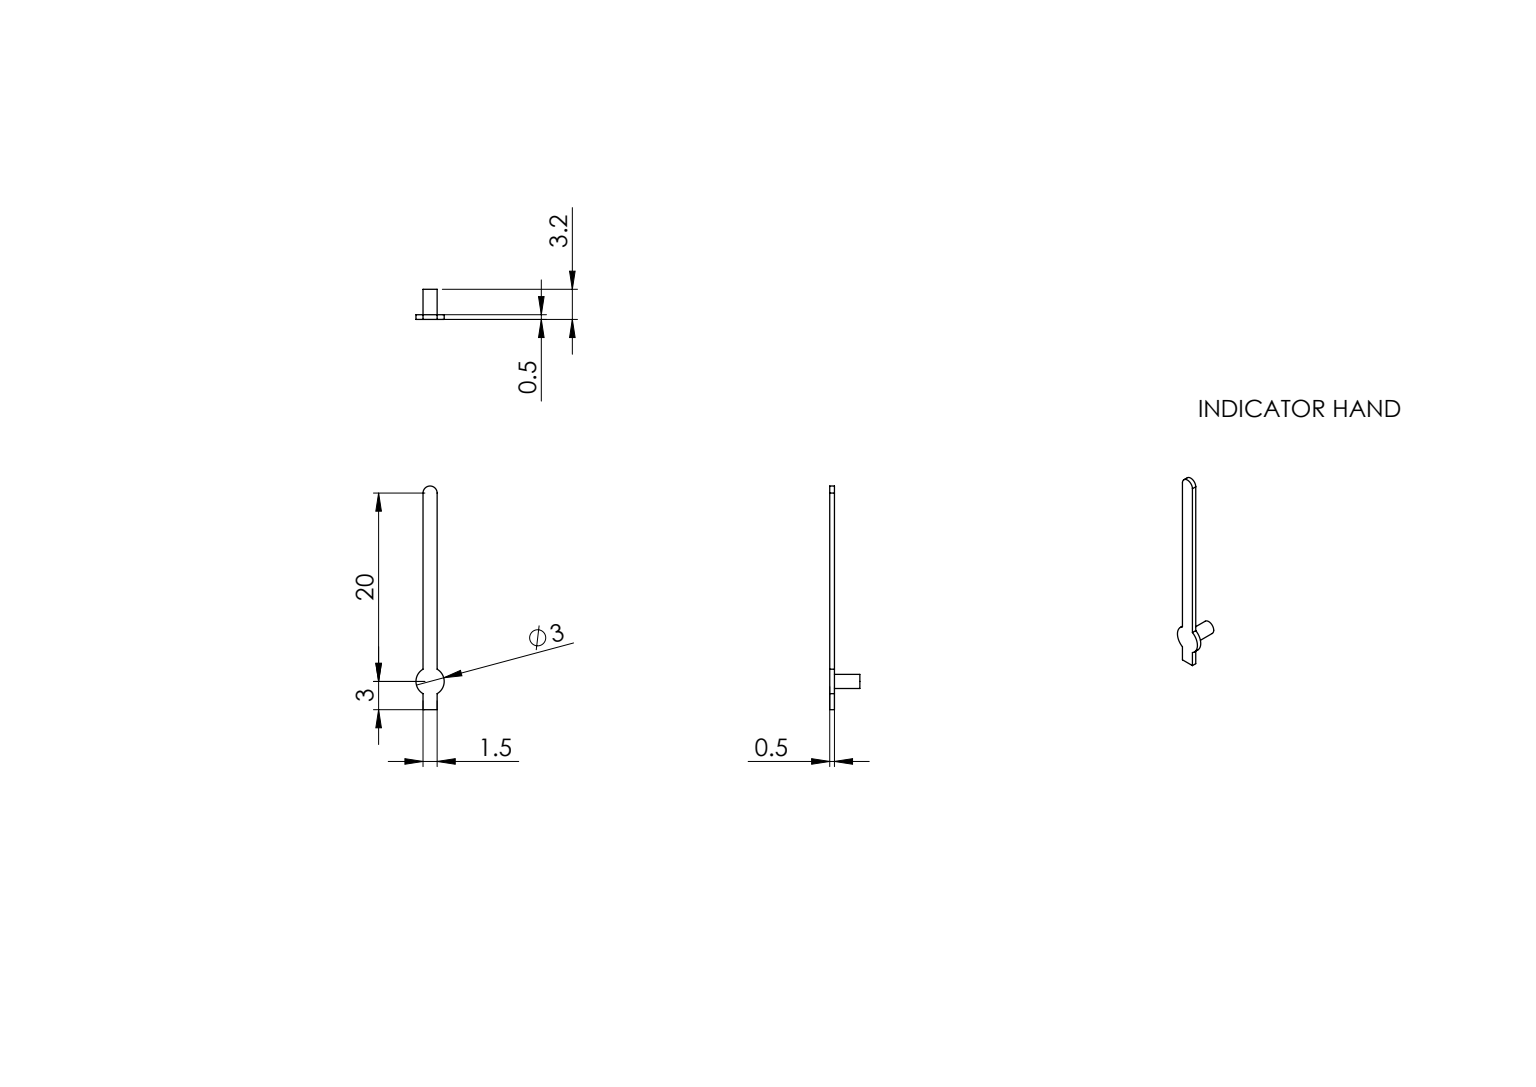
ISO-10303-21;
HEADER;
FILE_DESCRIPTION (('STEP AP214'),
    '1' );
FILE_NAME ('indicator hand.step',
    '2026-10-26T12:50:16',
    ( '' ),
    ( '' ),
    'SwSTEP 2.0',
    'SolidWorks 2026',
    '' );
FILE_SCHEMA (( 'AUTOMOTIVE_DESIGN' ));
ENDSEC;

DATA;
#4=SHAPE_REPRESENTATION_RELATIONSHIP ( 'NONE' , 'NONE' ,  #4483, #7868 ) ;
#16=EDGE_CURVE ( 'NONE', #18357, #14663, #23368, .T. ) ;
#30=CYLINDRICAL_SURFACE ( 'NONE', #8395, 1.500000000000000222 ) ;
#77=( LENGTH_UNIT ( ) NAMED_UNIT ( * ) SI_UNIT ( .MILLI., .METRE. ) );
#128=LINE ( 'NONE', #11881, #5846 ) ;
#265=DIRECTION ( 'NONE',  ( -0.000000000000000000, 0.000000000000000000, 1.000000000000000000 ) ) ;
#311=VERTEX_POINT ( 'NONE', #18646 ) ;
#314=EDGE_CURVE ( 'NONE', #21568, #311, #8696, .T. ) ;
#316=ORIENTED_EDGE ( 'NONE', *, *, #23479, .F. ) ;
#369=ORIENTED_EDGE ( 'NONE', *, *, #4197, .F. ) ;
#391=DIRECTION ( 'NONE',  ( 0.000000000000000000, 0.000000000000000000, -1.000000000000000000 ) ) ;
#413=CIRCLE ( 'NONE', #7088, 1.500000000000000222 ) ;
#423=LINE ( 'NONE', #3954, #1333 ) ;
#454=ORIENTED_EDGE ( 'NONE', *, *, #18989, .T. ) ;
#496=PLANE ( 'NONE',  #9182 ) ;
#529=SURFACE_STYLE_FILL_AREA ( #10305 ) ;
#580=ORIENTED_EDGE ( 'NONE', *, *, #2262, .F. ) ;
#760=ORIENTED_EDGE ( 'NONE', *, *, #22579, .T. ) ;
#774=UNCERTAINTY_MEASURE_WITH_UNIT (LENGTH_MEASURE( 1.000000000000000082E-05 ), #11385, 'distance_accuracy_value', 'NONE');
#973=AXIS2_PLACEMENT_3D ( 'NONE', #20831, #5152, #18742 ) ;
#1217=AXIS2_PLACEMENT_3D ( 'NONE', #13567, #5586, #21034 ) ;
#1245=AXIS2_PLACEMENT_3D ( 'NONE', #6493, #22719, #12504 ) ;
#1333=VECTOR ( 'NONE', #12312, 1000.000000000000000 ) ;
#1367=EDGE_CURVE ( 'NONE', #19382, #4582, #423, .T. ) ;
#1374=ORIENTED_EDGE ( 'NONE', *, *, #24355, .F. ) ;
#1437=CARTESIAN_POINT ( 'NONE',  ( -0.7500000000000001110, 20.00000000000000000, 18.19999999999999929 ) ) ;
#1466=ADVANCED_FACE ( 'NONE', ( #12569 ), #4854, .T. ) ;
#1469=DIRECTION ( 'NONE',  ( 1.000000000000000000, 0.000000000000000000, 0.000000000000000000 ) ) ;
#1552=LINE ( 'NONE', #23523, #5088 ) ;
#1604=VECTOR ( 'NONE', #22634, 1000.000000000000000 ) ;
#1679=CYLINDRICAL_SURFACE ( 'NONE', #11711, 0.7500000000000001110 ) ;
#1751=VECTOR ( 'NONE', #15740, 1000.000000000000000 ) ;
#1825=STYLED_ITEM ( 'NONE', ( #22348 ), #7868 ) ;
#1862=ORIENTED_EDGE ( 'NONE', *, *, #1367, .F. ) ;
#1894=VERTEX_POINT ( 'NONE', #17356 ) ;
#1944=DIRECTION ( 'NONE',  ( 1.000000000000000000, 0.000000000000000000, 0.000000000000000000 ) ) ;
#2058=CARTESIAN_POINT ( 'NONE',  ( -0.7500000000000001110, 20.00000000000000000, 17.69999999999999929 ) ) ;
#2084=CARTESIAN_POINT ( 'NONE',  ( 0.000000000000000000, 20.00000000000000000, 18.19999999999999929 ) ) ;
#2140=CARTESIAN_POINT ( 'NONE',  ( 0.7500000000000000000, -1.299038105676658450, 17.69999999999999929 ) ) ;
#2150=ORIENTED_EDGE ( 'NONE', *, *, #3374, .T. ) ;
#2219=EDGE_LOOP ( 'NONE', ( #9954, #6871, #760, #24291 ) ) ;
#2246=LINE ( 'NONE', #10201, #8730 ) ;
#2262=EDGE_CURVE ( 'NONE', #15216, #21568, #413, .T. ) ;
#2396=CARTESIAN_POINT ( 'NONE',  ( -0.7500000000000000000, -2.999999999999999556, 17.69999999999999929 ) ) ;
#2437=CARTESIAN_POINT ( 'NONE',  ( 0.000000000000000000, 0.000000000000000000, 17.69999999999999929 ) ) ;
#2546=PRODUCT ( 'indicator hand', 'indicator hand', '', ( #13281 ) ) ;
#2551=VECTOR ( 'NONE', #23517, 1000.000000000000000 ) ;
#2557=ORIENTED_EDGE ( 'NONE', *, *, #11543, .T. ) ;
#2590=AXIS2_PLACEMENT_3D ( 'NONE', #24800, #12151, #265 ) ;
#2619=CARTESIAN_POINT ( 'NONE',  ( -0.7500000000000001110, 0.000000000000000000, 17.69999999999999929 ) ) ;
#2630=ADVANCED_FACE ( 'NONE', ( #4724 ), #21062, .T. ) ;
#2824=EDGE_CURVE ( 'NONE', #1894, #20362, #128, .T. ) ;
#3021=ORIENTED_EDGE ( 'NONE', *, *, #17150, .F. ) ;
#3025=VERTEX_POINT ( 'NONE', #18252 ) ;
#3077=VERTEX_POINT ( 'NONE', #13150 ) ;
#3241=DIRECTION ( 'NONE',  ( -0.000000000000000000, -0.000000000000000000, -1.000000000000000000 ) ) ;
#3374=EDGE_CURVE ( 'NONE', #4582, #7827, #4205, .T. ) ;
#3456=EDGE_CURVE ( 'NONE', #24553, #20362, #14318, .T. ) ;
#3553=ORIENTED_EDGE ( 'NONE', *, *, #20988, .F. ) ;
#3588=FACE_OUTER_BOUND ( 'NONE', #25625, .T. ) ;
#3618=EDGE_LOOP ( 'NONE', ( #580, #15779, #14975, #18678, #23631, #13884, #15664, #1862, #21241 ) ) ;
#3631=CARTESIAN_POINT ( 'NONE',  ( 0.000000000000000000, 0.000000000000000000, 18.19999999999999929 ) ) ;
#3637=DIRECTION ( 'NONE',  ( 0.000000000000000000, 0.000000000000000000, 1.000000000000000000 ) ) ;
#3655=( NAMED_UNIT ( * ) SI_UNIT ( $, .STERADIAN. ) SOLID_ANGLE_UNIT ( ) );
#3716=AXIS2_PLACEMENT_3D ( 'NONE', #17008, #23151, #11229 ) ;
#3846=ORIENTED_EDGE ( 'NONE', *, *, #6041, .F. ) ;
#3864=CARTESIAN_POINT ( 'NONE',  ( -0.7500000000000001110, 0.000000000000000000, 15.00000000000000178 ) ) ;
#3938=ADVANCED_FACE ( 'NONE', ( #19773 ), #30, .T. ) ;
#3954=CARTESIAN_POINT ( 'NONE',  ( 0.7500000000000001110, 0.000000000000000000, 17.69999999999999929 ) ) ;
#4014=DIRECTION ( 'NONE',  ( -0.000000000000000000, -0.000000000000000000, -1.000000000000000000 ) ) ;
#4109=VECTOR ( 'NONE', #3241, 1000.000000000000000 ) ;
#4197=EDGE_CURVE ( 'NONE', #3025, #1894, #12706, .T. ) ;
#4205=CIRCLE ( 'NONE', #8806, 0.7500000000000001110 ) ;
#4304=EDGE_LOOP ( 'NONE', ( #7201, #7831, #1374, #13092 ) ) ;
#4430=EDGE_CURVE ( 'NONE', #25396, #19442, #11352, .T. ) ;
#4452=ORIENTED_EDGE ( 'NONE', *, *, #3456, .T. ) ;
#4483=SHAPE_REPRESENTATION ( 'indicator hand', ( #21036 ), #24374 ) ;
#4486=LINE ( 'NONE', #14704, #7644 ) ;
#4550=ORIENTED_EDGE ( 'NONE', *, *, #23479, .T. ) ;
#4572=CARTESIAN_POINT ( 'NONE',  ( -0.7500000000000000000, 0.000000000000000000, 18.19999999999999929 ) ) ;
#4582=VERTEX_POINT ( 'NONE', #15817 ) ;
#4587=CIRCLE ( 'NONE', #1245, 0.7500000000000001110 ) ;
#4612=EDGE_CURVE ( 'NONE', #3077, #15986, #23092, .T. ) ;
#4645=ORIENTED_EDGE ( 'NONE', *, *, #23598, .T. ) ;
#4666=FACE_OUTER_BOUND ( 'NONE', #3618, .T. ) ;
#4707=DIRECTION ( 'NONE',  ( -0.000000000000000000, -1.000000000000000000, 0.000000000000000000 ) ) ;
#4724=FACE_OUTER_BOUND ( 'NONE', #5151, .T. ) ;
#4764=ORIENTED_EDGE ( 'NONE', *, *, #12435, .F. ) ;
#4854=CYLINDRICAL_SURFACE ( 'NONE', #24875, 1.500000000000000222 ) ;
#4858=DIRECTION ( 'NONE',  ( 0.000000000000000000, 0.000000000000000000, 1.000000000000000000 ) ) ;
#4912=CARTESIAN_POINT ( 'NONE',  ( 0.7500000000000001110, 0.000000000000000000, 17.69999999999999929 ) ) ;
#4913=CARTESIAN_POINT ( 'NONE',  ( 0.7500000000000001110, 1.299038105676658450, 17.69999999999999929 ) ) ;
#5050=ADVANCED_FACE ( 'NONE', ( #3588 ), #25691, .T. ) ;
#5088=VECTOR ( 'NONE', #9520, 1000.000000000000000 ) ;
#5094=AXIS2_PLACEMENT_3D ( 'NONE', #11723, #9768, #14441 ) ;
#5142=EDGE_CURVE ( 'NONE', #19442, #3077, #4486, .T. ) ;
#5151=EDGE_LOOP ( 'NONE', ( #9902, #23149, #17711, #4452 ) ) ;
#5152=DIRECTION ( 'NONE',  ( -0.000000000000000000, -0.000000000000000000, -1.000000000000000000 ) ) ;
#5159=DIRECTION ( 'NONE',  ( 0.000000000000000000, 0.000000000000000000, 1.000000000000000000 ) ) ;
#5272=ADVANCED_FACE ( 'NONE', ( #9680 ), #13723, .T. ) ;
#5355=VERTEX_POINT ( 'NONE', #23664 ) ;
#5405=STYLED_ITEM('',(#25907),#13235);
#5417=AXIS2_PLACEMENT_3D ( 'NONE', #17332, #19276, #17062 ) ;
#5453=AXIS2_PLACEMENT_3D ( 'NONE', #7275, #15251, #17705 ) ;
#5586=DIRECTION ( 'NONE',  ( 0.000000000000000000, 0.000000000000000000, 1.000000000000000000 ) ) ;
#5588=( GEOMETRIC_REPRESENTATION_CONTEXT ( 3 ) GLOBAL_UNCERTAINTY_ASSIGNED_CONTEXT ( ( #16739 ) ) GLOBAL_UNIT_ASSIGNED_CONTEXT ( ( #16351, #10186, #6015 ) ) REPRESENTATION_CONTEXT ( 'NONE', 'WORKASPACE' ) );
#5739=ORIENTED_EDGE ( 'NONE', *, *, #4430, .F. ) ;
#5774=CARTESIAN_POINT ( 'NONE',  ( 0.7500000000000001110, 20.00000000000000000, 18.19999999999999929 ) ) ;
#5846=VECTOR ( 'NONE', #23777, 1000.000000000000000 ) ;
#5872=VERTEX_POINT ( 'NONE', #13031 ) ;
#5909=CIRCLE ( 'NONE', #17198, 1.500000000000000222 ) ;
#6015=( NAMED_UNIT ( * ) SI_UNIT ( $, .STERADIAN. ) SOLID_ANGLE_UNIT ( ) );
#6041=EDGE_CURVE ( 'NONE', #5355, #311, #5909, .T. ) ;
#6064=CARTESIAN_POINT ( 'NONE',  ( 0.000000000000000000, 20.00000000000000000, 17.69999999999999929 ) ) ;
#6175=CARTESIAN_POINT ( 'NONE',  ( -0.7500000000000000000, -2.999999999999999556, 17.69999999999999929 ) ) ;
#6390=ORIENTED_EDGE ( 'NONE', *, *, #5142, .T. ) ;
#6404=AXIS2_PLACEMENT_3D ( 'NONE', #21077, #4858, #23164 ) ;
#6484=ORIENTED_EDGE ( 'NONE', *, *, #9563, .T. ) ;
#6493=CARTESIAN_POINT ( 'NONE',  ( 0.000000000000000000, 0.000000000000000000, 15.00000000000000178 ) ) ;
#6585=ADVANCED_FACE ( 'NONE', ( #14390 ), #16837, .F. ) ;
#6588=ADVANCED_FACE ( 'NONE', ( #22839 ), #20125, .T. ) ;
#6709=DIRECTION ( 'NONE',  ( -0.000000000000000000, -1.000000000000000000, -0.000000000000000000 ) ) ;
#6742=ORIENTED_EDGE ( 'NONE', *, *, #14143, .F. ) ;
#6755=FACE_BOUND ( 'NONE', #21088, .T. ) ;
#6783=DIRECTION ( 'NONE',  ( 0.000000000000000000, 0.000000000000000000, 1.000000000000000000 ) ) ;
#6812=ORIENTED_EDGE ( 'NONE', *, *, #23697, .F. ) ;
#6822=EDGE_CURVE ( 'NONE', #21568, #19382, #7180, .T. ) ;
#6871=ORIENTED_EDGE ( 'NONE', *, *, #6822, .T. ) ;
#6901=EDGE_LOOP ( 'NONE', ( #23596, #22832, #7859, #24550, #11914, #10464, #7157, #23330, #6390 ) ) ;
#7058=PLANE ( 'NONE',  #3716 ) ;
#7073=CARTESIAN_POINT ( 'NONE',  ( 0.7500000000000001110, 1.299038105676658450, 18.19999999999999929 ) ) ;
#7088=AXIS2_PLACEMENT_3D ( 'NONE', #20724, #10767, #1469 ) ;
#7112=CARTESIAN_POINT ( 'NONE',  ( 0.000000000000000000, 0.000000000000000000, 17.69999999999999929 ) ) ;
#7157=ORIENTED_EDGE ( 'NONE', *, *, #23697, .T. ) ;
#7180=CIRCLE ( 'NONE', #5094, 1.500000000000000222 ) ;
#7201=ORIENTED_EDGE ( 'NONE', *, *, #2824, .T. ) ;
#7275=CARTESIAN_POINT ( 'NONE',  ( 0.000000000000000000, 0.000000000000000000, 15.00000000000000178 ) ) ;
#7347=DIRECTION ( 'NONE',  ( 0.000000000000000000, 0.000000000000000000, 1.000000000000000000 ) ) ;
#7469=VECTOR ( 'NONE', #7347, 1000.000000000000000 ) ;
#7556=VECTOR ( 'NONE', #22573, 1000.000000000000000 ) ;
#7616=EDGE_LOOP ( 'NONE', ( #20823, #18587, #4645, #21349 ) ) ;
#7644=VECTOR ( 'NONE', #6709, 1000.000000000000000 ) ;
#7690=PRODUCT_DEFINITION_FORMATION_WITH_SPECIFIED_SOURCE ( 'ANY', '', #2546, .NOT_KNOWN. ) ;
#7827=VERTEX_POINT ( 'NONE', #22485 ) ;
#7831=ORIENTED_EDGE ( 'NONE', *, *, #3456, .F. ) ;
#7859=ORIENTED_EDGE ( 'NONE', *, *, #2824, .F. ) ;
#7868=ADVANCED_BREP_SHAPE_REPRESENTATION ( '', ( #13235, #21036 ), #24374 ) ;
#7879=LINE ( 'NONE', #23839, #1751 ) ;
#7943=CARTESIAN_POINT ( 'NONE',  ( 0.000000000000000000, 0.000000000000000000, 15.00000000000000178 ) ) ;
#7958=ORIENTED_EDGE ( 'NONE', *, *, #1367, .T. ) ;
#7999=VECTOR ( 'NONE', #22720, 1000.000000000000000 ) ;
#8023=VECTOR ( 'NONE', #14665, 1000.000000000000000 ) ;
#8108=DIRECTION ( 'NONE',  ( 1.000000000000000000, 0.000000000000000000, 0.000000000000000000 ) ) ;
#8137=DIRECTION ( 'NONE',  ( 0.000000000000000000, 0.000000000000000000, 1.000000000000000000 ) ) ;
#8355=DIRECTION ( 'NONE',  ( 1.000000000000000000, 0.000000000000000000, 0.000000000000000000 ) ) ;
#8395=AXIS2_PLACEMENT_3D ( 'NONE', #12176, #8137, #13754 ) ;
#8417=CARTESIAN_POINT ( 'NONE',  ( -0.7500000000000000000, -2.999999999999999556, 18.19999999999999929 ) ) ;
#8696=LINE ( 'NONE', #22955, #7556 ) ;
#8730=VECTOR ( 'NONE', #16227, 1000.000000000000000 ) ;
#8806=AXIS2_PLACEMENT_3D ( 'NONE', #6064, #12067, #16017 ) ;
#8848=VECTOR ( 'NONE', #4707, 1000.000000000000000 ) ;
#8854=DIRECTION ( 'NONE',  ( 1.000000000000000000, 0.000000000000000000, -0.000000000000000000 ) ) ;
#8916=ORIENTED_EDGE ( 'NONE', *, *, #10895, .T. ) ;
#9078=FACE_OUTER_BOUND ( 'NONE', #9251, .T. ) ;
#9106=AXIS2_PLACEMENT_3D ( 'NONE', #20134, #9934, #25645 ) ;
#9131=UNCERTAINTY_MEASURE_WITH_UNIT (LENGTH_MEASURE( 1.000000000000000082E-05 ), #77, 'distance_accuracy_value', 'NONE');
#9182=AXIS2_PLACEMENT_3D ( 'NONE', #2437, #14603, #8854 ) ;
#9251=EDGE_LOOP ( 'NONE', ( #5739, #20270, #2150, #12563 ) ) ;
#9316=LINE ( 'NONE', #25266, #7469 ) ;
#9351=CYLINDRICAL_SURFACE ( 'NONE', #5417, 0.7500000000000001110 ) ;
#9513=LINE ( 'NONE', #23008, #2551 ) ;
#9520=DIRECTION ( 'NONE',  ( -0.000000000000000000, -0.000000000000000000, -1.000000000000000000 ) ) ;
#9563=EDGE_CURVE ( 'NONE', #15156, #20673, #11282, .T. ) ;
#9565=CARTESIAN_POINT ( 'NONE',  ( -0.7500000000000000000, -1.299038105676658450, 17.69999999999999929 ) ) ;
#9680=FACE_OUTER_BOUND ( 'NONE', #23184, .T. ) ;
#9768=DIRECTION ( 'NONE',  ( 0.000000000000000000, 0.000000000000000000, 1.000000000000000000 ) ) ;
#9821=PRODUCT_DEFINITION ( 'UNKNOWN', '', #7690, #23252 ) ;
#9902=ORIENTED_EDGE ( 'NONE', *, *, #15885, .F. ) ;
#9934=DIRECTION ( 'NONE',  ( 0.000000000000000000, 1.000000000000000000, -0.000000000000000000 ) ) ;
#9954=ORIENTED_EDGE ( 'NONE', *, *, #314, .F. ) ;
#10021=LINE ( 'NONE', #2058, #25053 ) ;
#10146=EDGE_CURVE ( 'NONE', #20673, #24553, #9513, .T. ) ;
#10186=( NAMED_UNIT ( * ) PLANE_ANGLE_UNIT ( ) SI_UNIT ( $, .RADIAN. ) );
#10201=CARTESIAN_POINT ( 'NONE',  ( -0.7500000000000000000, -1.299038105676658450, 17.69999999999999929 ) ) ;
#10305=FILL_AREA_STYLE ('',( #12153 ) ) ;
#10464=ORIENTED_EDGE ( 'NONE', *, *, #25796, .T. ) ;
#10689=PRODUCT_DEFINITION_SHAPE ( 'NONE', 'NONE',  #9821 ) ;
#10722=CARTESIAN_POINT ( 'NONE',  ( 0.000000000000000000, 0.000000000000000000, 17.69999999999999929 ) ) ;
#10757=CARTESIAN_POINT ( 'NONE',  ( 1.500000000000000222, 0.000000000000000000, 17.69999999999999929 ) ) ;
#10767=DIRECTION ( 'NONE',  ( 0.000000000000000000, 0.000000000000000000, 1.000000000000000000 ) ) ;
#10891=VECTOR ( 'NONE', #4014, 1000.000000000000000 ) ;
#10895=EDGE_CURVE ( 'NONE', #7827, #15156, #21821, .T. ) ;
#10941=AXIS2_PLACEMENT_3D ( 'NONE', #2084, #23662, #8108 ) ;
#10996=DIRECTION ( 'NONE',  ( 1.000000000000000000, 0.000000000000000000, 0.000000000000000000 ) ) ;
#11107=DIRECTION ( 'NONE',  ( -1.000000000000000000, 0.000000000000000000, -0.000000000000000000 ) ) ;
#11229=DIRECTION ( 'NONE',  ( 1.000000000000000000, 0.000000000000000000, -0.000000000000000000 ) ) ;
#11282=CIRCLE ( 'NONE', #14636, 1.500000000000000222 ) ;
#11352=CIRCLE ( 'NONE', #10941, 0.7500000000000001110 ) ;
#11368=CARTESIAN_POINT ( 'NONE',  ( -0.7500000000000000000, 0.000000000000000000, 17.69999999999999929 ) ) ;
#11385=( LENGTH_UNIT ( ) NAMED_UNIT ( * ) SI_UNIT ( .MILLI., .METRE. ) );
#11398=AXIS2_PLACEMENT_3D ( 'NONE', #21767, #19668, #22017 ) ;
#11407=ORIENTED_EDGE ( 'NONE', *, *, #13065, .F. ) ;
#11425=MECHANICAL_DESIGN_GEOMETRIC_PRESENTATION_REPRESENTATION('',(#1825),#5588);
#11509=( NAMED_UNIT ( * ) PLANE_ANGLE_UNIT ( ) SI_UNIT ( $, .RADIAN. ) );
#11526=ORIENTED_EDGE ( 'NONE', *, *, #20988, .T. ) ;
#11543=EDGE_CURVE ( 'NONE', #5355, #1894, #16288, .T. ) ;
#11586=DIRECTION ( 'NONE',  ( -0.000000000000000000, -0.000000000000000000, -1.000000000000000000 ) ) ;
#11711=AXIS2_PLACEMENT_3D ( 'NONE', #3631, #17380, #19335 ) ;
#11723=CARTESIAN_POINT ( 'NONE',  ( 0.000000000000000000, 0.000000000000000000, 17.69999999999999929 ) ) ;
#11807=AXIS2_PLACEMENT_3D ( 'NONE', #22344, #6783, #8355 ) ;
#11876=CARTESIAN_POINT ( 'NONE',  ( 0.000000000000000000, 0.000000000000000000, 17.69999999999999929 ) ) ;
#11881=CARTESIAN_POINT ( 'NONE',  ( 0.7500000000000000000, -2.999999999999999556, 18.19999999999999929 ) ) ;
#11914=ORIENTED_EDGE ( 'NONE', *, *, #6041, .T. ) ;
#11927=SHAPE_DEFINITION_REPRESENTATION ( #10689, #4483 ) ;
#12067=DIRECTION ( 'NONE',  ( 0.000000000000000000, 0.000000000000000000, 1.000000000000000000 ) ) ;
#12079=DIRECTION ( 'NONE',  ( 0.000000000000000000, 0.000000000000000000, 1.000000000000000000 ) ) ;
#12151=DIRECTION ( 'NONE',  ( -1.000000000000000000, 0.000000000000000000, -0.000000000000000000 ) ) ;
#12153=FILL_AREA_STYLE_COLOUR ( '', #13100 ) ;
#12176=CARTESIAN_POINT ( 'NONE',  ( 0.000000000000000000, 0.000000000000000000, 17.69999999999999929 ) ) ;
#12312=DIRECTION ( 'NONE',  ( 0.000000000000000000, 1.000000000000000000, 0.000000000000000000 ) ) ;
#12435=EDGE_CURVE ( 'NONE', #15216, #3025, #14124, .T. ) ;
#12504=DIRECTION ( 'NONE',  ( 1.000000000000000000, 0.000000000000000000, 0.000000000000000000 ) ) ;
#12505=LINE ( 'NONE', #20620, #7999 ) ;
#12563=ORIENTED_EDGE ( 'NONE', *, *, #22316, .T. ) ;
#12569=FACE_OUTER_BOUND ( 'NONE', #2219, .T. ) ;
#12694=CARTESIAN_POINT ( 'NONE',  ( 0.7500000000000001110, 1.299038105676658450, 17.69999999999999929 ) ) ;
#12706=LINE ( 'NONE', #14529, #8023 ) ;
#12727=EDGE_LOOP ( 'NONE', ( #11407, #23431 ) ) ;
#12995=ADVANCED_FACE ( 'NONE', ( #4666, #6755 ), #496, .F. ) ;
#13031=CARTESIAN_POINT ( 'NONE',  ( 0.7500000000000001110, 9.184850993605150903E-17, 15.00000000000000178 ) ) ;
#13065=EDGE_CURVE ( 'NONE', #14663, #5872, #4587, .T. ) ;
#13091=EDGE_LOOP ( 'NONE', ( #3021, #19791, #19901, #6484 ) ) ;
#13092=ORIENTED_EDGE ( 'NONE', *, *, #4197, .T. ) ;
#13100=COLOUR_RGB ( '',0.8941176470588234615, 0.8941176470588234615, 0.8941176470588234615 ) ;
#13136=DIRECTION ( 'NONE',  ( 1.000000000000000000, 0.000000000000000000, 0.000000000000000000 ) ) ;
#13150=CARTESIAN_POINT ( 'NONE',  ( -0.7500000000000001110, 1.299038105676658450, 18.19999999999999929 ) ) ;
#13223=DIRECTION ( 'NONE',  ( 1.000000000000000000, 0.000000000000000000, 0.000000000000000000 ) ) ;
#13235=MANIFOLD_SOLID_BREP ( 'Extrude-Thin1', #17985 ) ;
#13281=PRODUCT_CONTEXT ( 'NONE', #15297, 'mechanical' ) ;
#13319=LINE ( 'NONE', #20220, #10891 ) ;
#13353=CARTESIAN_POINT ( 'NONE',  ( 0.000000000000000000, 0.000000000000000000, 0.000000000000000000 ) ) ;
#13369=EDGE_LOOP ( 'NONE', ( #20328, #7958, #454, #6812 ) ) ;
#13567=CARTESIAN_POINT ( 'NONE',  ( 0.000000000000000000, 0.000000000000000000, 17.69999999999999929 ) ) ;
#13723=CYLINDRICAL_SURFACE ( 'NONE', #973, 0.7500000000000001110 ) ;
#13754=DIRECTION ( 'NONE',  ( 1.000000000000000000, 0.000000000000000000, 0.000000000000000000 ) ) ;
#13876=PLANE ( 'NONE',  #9106 ) ;
#13884=ORIENTED_EDGE ( 'NONE', *, *, #10895, .F. ) ;
#14061=ADVANCED_FACE ( 'NONE', ( #17638 ), #1679, .T. ) ;
#14124=LINE ( 'NONE', #22089, #8848 ) ;
#14143=EDGE_CURVE ( 'NONE', #3077, #15156, #19197, .T. ) ;
#14258=DIRECTION ( 'NONE',  ( 1.000000000000000000, 0.000000000000000000, 0.000000000000000000 ) ) ;
#14260=SURFACE_SIDE_STYLE ('',( #529 ) ) ;
#14277=ORIENTED_EDGE ( 'NONE', *, *, #5142, .F. ) ;
#14318=LINE ( 'NONE', #2396, #16747 ) ;
#14390=FACE_OUTER_BOUND ( 'NONE', #18611, .T. ) ;
#14441=DIRECTION ( 'NONE',  ( 1.000000000000000000, 0.000000000000000000, 0.000000000000000000 ) ) ;
#14456=DIRECTION ( 'NONE',  ( -0.000000000000000000, -1.000000000000000000, 0.000000000000000000 ) ) ;
#14529=CARTESIAN_POINT ( 'NONE',  ( 0.7500000000000000000, -2.999999999999999556, 17.69999999999999929 ) ) ;
#14603=DIRECTION ( 'NONE',  ( 0.000000000000000000, 0.000000000000000000, 1.000000000000000000 ) ) ;
#14636=AXIS2_PLACEMENT_3D ( 'NONE', #7112, #5159, #13136 ) ;
#14663=VERTEX_POINT ( 'NONE', #3864 ) ;
#14665=DIRECTION ( 'NONE',  ( 0.000000000000000000, 0.000000000000000000, 1.000000000000000000 ) ) ;
#14704=CARTESIAN_POINT ( 'NONE',  ( -0.7500000000000001110, 0.000000000000000000, 18.19999999999999929 ) ) ;
#14792=FACE_OUTER_BOUND ( 'NONE', #6901, .T. ) ;
#14975=ORIENTED_EDGE ( 'NONE', *, *, #24355, .T. ) ;
#15080=ORIENTED_EDGE ( 'NONE', *, *, #22316, .F. ) ;
#15156=VERTEX_POINT ( 'NONE', #23079 ) ;
#15182=DIRECTION ( 'NONE',  ( -0.000000000000000000, 0.000000000000000000, 1.000000000000000000 ) ) ;
#15216=VERTEX_POINT ( 'NONE', #2140 ) ;
#15251=DIRECTION ( 'NONE',  ( 0.000000000000000000, 0.000000000000000000, 1.000000000000000000 ) ) ;
#15271=ORIENTED_EDGE ( 'NONE', *, *, #13065, .T. ) ;
#15297=APPLICATION_CONTEXT ( 'automotive_design' ) ;
#15450=APPLICATION_CONTEXT ( 'automotive_design' ) ;
#15484=VECTOR ( 'NONE', #11586, 1000.000000000000000 ) ;
#15664=ORIENTED_EDGE ( 'NONE', *, *, #3374, .F. ) ;
#15703=DIRECTION ( 'NONE',  ( 0.000000000000000000, 0.000000000000000000, 1.000000000000000000 ) ) ;
#15704=EDGE_CURVE ( 'NONE', #20366, #18357, #19125, .T. ) ;
#15736=PLANE ( 'NONE',  #5453 ) ;
#15740=DIRECTION ( 'NONE',  ( -1.000000000000000000, 0.000000000000000000, 0.000000000000000000 ) ) ;
#15779=ORIENTED_EDGE ( 'NONE', *, *, #12435, .T. ) ;
#15799=DIRECTION ( 'NONE',  ( -0.000000000000000000, -1.000000000000000000, -0.000000000000000000 ) ) ;
#15817=CARTESIAN_POINT ( 'NONE',  ( 0.7500000000000001110, 20.00000000000000000, 17.69999999999999929 ) ) ;
#15885=EDGE_CURVE ( 'NONE', #15986, #20362, #22359, .T. ) ;
#15930=DIRECTION ( 'NONE',  ( 0.000000000000000000, 0.000000000000000000, 1.000000000000000000 ) ) ;
#15965=SURFACE_STYLE_USAGE ( .BOTH. , #14260 ) ;
#15980=CARTESIAN_POINT ( 'NONE',  ( 0.000000000000000000, 0.000000000000000000, 17.69999999999999929 ) ) ;
#15986=VERTEX_POINT ( 'NONE', #22238 ) ;
#16017=DIRECTION ( 'NONE',  ( 1.000000000000000000, 0.000000000000000000, 0.000000000000000000 ) ) ;
#16207=ADVANCED_FACE ( 'NONE', ( #17506 ), #19583, .T. ) ;
#16227=DIRECTION ( 'NONE',  ( -0.000000000000000000, -0.000000000000000000, -1.000000000000000000 ) ) ;
#16288=LINE ( 'NONE', #24393, #20529 ) ;
#16351=( LENGTH_UNIT ( ) NAMED_UNIT ( * ) SI_UNIT ( .MILLI., .METRE. ) );
#16511=DIRECTION ( 'NONE',  ( 0.000000000000000000, 0.000000000000000000, 1.000000000000000000 ) ) ;
#16739=UNCERTAINTY_MEASURE_WITH_UNIT (LENGTH_MEASURE( 1.000000000000000082E-05 ), #16351, 'distance_accuracy_value', 'NONE');
#16747=VECTOR ( 'NONE', #18734, 1000.000000000000000 ) ;
#16781=CIRCLE ( 'NONE', #20093, 0.7500000000000001110 ) ;
#16788=AXIS2_PLACEMENT_3D ( 'NONE', #4912, #14258, #391 ) ;
#16837=PLANE ( 'NONE',  #2590 ) ;
#17008=CARTESIAN_POINT ( 'NONE',  ( 0.000000000000000000, 0.000000000000000000, 18.19999999999999929 ) ) ;
#17062=DIRECTION ( 'NONE',  ( 1.000000000000000000, 0.000000000000000000, 0.000000000000000000 ) ) ;
#17150=EDGE_CURVE ( 'NONE', #15986, #20673, #2246, .T. ) ;
#17198=AXIS2_PLACEMENT_3D ( 'NONE', #20054, #12079, #17848 ) ;
#17223=FACE_OUTER_BOUND ( 'NONE', #12727, .T. ) ;
#17312=ADVANCED_FACE ( 'NONE', ( #14792 ), #7058, .T. ) ;
#17332=CARTESIAN_POINT ( 'NONE',  ( 0.000000000000000000, 20.00000000000000000, 17.69999999999999929 ) ) ;
#17356=CARTESIAN_POINT ( 'NONE',  ( 0.7500000000000000000, -2.999999999999999556, 18.19999999999999929 ) ) ;
#17380=DIRECTION ( 'NONE',  ( -0.000000000000000000, -0.000000000000000000, -1.000000000000000000 ) ) ;
#17506=FACE_OUTER_BOUND ( 'NONE', #25628, .T. ) ;
#17638=FACE_OUTER_BOUND ( 'NONE', #7616, .T. ) ;
#17681=DIRECTION ( 'NONE',  ( 0.000000000000000000, 0.000000000000000000, 1.000000000000000000 ) ) ;
#17705=DIRECTION ( 'NONE',  ( 1.000000000000000000, 0.000000000000000000, -0.000000000000000000 ) ) ;
#17711=ORIENTED_EDGE ( 'NONE', *, *, #10146, .T. ) ;
#17848=DIRECTION ( 'NONE',  ( 1.000000000000000000, 0.000000000000000000, 0.000000000000000000 ) ) ;
#17985=CLOSED_SHELL ( 'NONE', ( #14061, #16207, #1466, #5272, #17312, #22565, #12995, #5050, #19985, #6588, #3938, #2630, #6585, #18181 ) ) ;
#18021=DIRECTION ( 'NONE',  ( 0.000000000000000000, 0.000000000000000000, 1.000000000000000000 ) ) ;
#18181=ADVANCED_FACE ( 'NONE', ( #19995 ), #13876, .F. ) ;
#18252=CARTESIAN_POINT ( 'NONE',  ( 0.7500000000000000000, -2.999999999999999556, 17.69999999999999929 ) ) ;
#18357=VERTEX_POINT ( 'NONE', #2619 ) ;
#18535=CIRCLE ( 'NONE', #6404, 1.500000000000000222 ) ;
#18559=ORIENTED_EDGE ( 'NONE', *, *, #2262, .T. ) ;
#18587=ORIENTED_EDGE ( 'NONE', *, *, #24712, .T. ) ;
#18611=EDGE_LOOP ( 'NONE', ( #316, #2557, #369, #4764 ) ) ;
#18646=CARTESIAN_POINT ( 'NONE',  ( 1.500000000000000222, 0.000000000000000000, 18.19999999999999929 ) ) ;
#18678=ORIENTED_EDGE ( 'NONE', *, *, #10146, .F. ) ;
#18734=DIRECTION ( 'NONE',  ( 0.000000000000000000, 0.000000000000000000, 1.000000000000000000 ) ) ;
#18742=DIRECTION ( 'NONE',  ( -1.000000000000000000, 0.000000000000000000, 0.000000000000000000 ) ) ;
#18753=ORIENTED_EDGE ( 'NONE', *, *, #24712, .F. ) ;
#18844=ORIENTED_EDGE ( 'NONE', *, *, #314, .T. ) ;
#18989=EDGE_CURVE ( 'NONE', #4582, #25396, #9316, .T. ) ;
#19125=CIRCLE ( 'NONE', #20369, 0.7500000000000001110 ) ;
#19197=LINE ( 'NONE', #21676, #4109 ) ;
#19248=ORIENTED_EDGE ( 'NONE', *, *, #15704, .T. ) ;
#19276=DIRECTION ( 'NONE',  ( 0.000000000000000000, 0.000000000000000000, 1.000000000000000000 ) ) ;
#19335=DIRECTION ( 'NONE',  ( -1.000000000000000000, 0.000000000000000000, 0.000000000000000000 ) ) ;
#19382=VERTEX_POINT ( 'NONE', #12694 ) ;
#19439=CARTESIAN_POINT ( 'NONE',  ( -0.7500000000000001110, 0.000000000000000000, 18.19999999999999929 ) ) ;
#19442=VERTEX_POINT ( 'NONE', #1437 ) ;
#19568=CIRCLE ( 'NONE', #1217, 0.7500000000000001110 ) ;
#19583=CYLINDRICAL_SURFACE ( 'NONE', #21639, 1.500000000000000222 ) ;
#19668=DIRECTION ( 'NONE',  ( -1.000000000000000000, 0.000000000000000000, 0.000000000000000000 ) ) ;
#19773=FACE_OUTER_BOUND ( 'NONE', #13091, .T. ) ;
#19791=ORIENTED_EDGE ( 'NONE', *, *, #4612, .F. ) ;
#19805=( NAMED_UNIT ( * ) PLANE_ANGLE_UNIT ( ) SI_UNIT ( $, .RADIAN. ) );
#19901=ORIENTED_EDGE ( 'NONE', *, *, #14143, .T. ) ;
#19985=ADVANCED_FACE ( 'NONE', ( #9078 ), #9351, .T. ) ;
#19995=FACE_OUTER_BOUND ( 'NONE', #4304, .T. ) ;
#20054=CARTESIAN_POINT ( 'NONE',  ( 0.000000000000000000, 0.000000000000000000, 18.19999999999999929 ) ) ;
#20093=AXIS2_PLACEMENT_3D ( 'NONE', #7943, #15930, #23761 ) ;
#20125=PLANE ( 'NONE',  #16788 ) ;
#20134=CARTESIAN_POINT ( 'NONE',  ( 0.7500000000000000000, -2.999999999999999556, 17.69999999999999929 ) ) ;
#20220=CARTESIAN_POINT ( 'NONE',  ( 0.7500000000000000000, -1.299038105676658450, 17.69999999999999929 ) ) ;
#20270=ORIENTED_EDGE ( 'NONE', *, *, #18989, .F. ) ;
#20300=CARTESIAN_POINT ( 'NONE',  ( 0.7500000000000001110, 9.184850993605150903E-17, 17.69999999999999929 ) ) ;
#20328=ORIENTED_EDGE ( 'NONE', *, *, #22579, .F. ) ;
#20362=VERTEX_POINT ( 'NONE', #8417 ) ;
#20366=VERTEX_POINT ( 'NONE', #20300 ) ;
#20369=AXIS2_PLACEMENT_3D ( 'NONE', #15980, #17681, #21978 ) ;
#20529=VECTOR ( 'NONE', #14456, 1000.000000000000000 ) ;
#20620=CARTESIAN_POINT ( 'NONE',  ( 0.7500000000000001110, 0.000000000000000000, 18.19999999999999929 ) ) ;
#20673=VERTEX_POINT ( 'NONE', #9565 ) ;
#20724=CARTESIAN_POINT ( 'NONE',  ( 0.000000000000000000, 0.000000000000000000, 17.69999999999999929 ) ) ;
#20823=ORIENTED_EDGE ( 'NONE', *, *, #15704, .F. ) ;
#20831=CARTESIAN_POINT ( 'NONE',  ( 0.000000000000000000, 0.000000000000000000, 18.19999999999999929 ) ) ;
#20872=DIRECTION ( 'NONE',  ( 0.000000000000000000, 0.000000000000000000, 1.000000000000000000 ) ) ;
#20988=EDGE_CURVE ( 'NONE', #18357, #20366, #19568, .T. ) ;
#21034=DIRECTION ( 'NONE',  ( 1.000000000000000000, 0.000000000000000000, 0.000000000000000000 ) ) ;
#21036=AXIS2_PLACEMENT_3D ( 'NONE', #13353, #15703, #13223 ) ;
#21062=PLANE ( 'NONE',  #23788 ) ;
#21077=CARTESIAN_POINT ( 'NONE',  ( 0.000000000000000000, 0.000000000000000000, 18.19999999999999929 ) ) ;
#21088=EDGE_LOOP ( 'NONE', ( #11526, #19248 ) ) ;
#21241=ORIENTED_EDGE ( 'NONE', *, *, #6822, .F. ) ;
#21349=ORIENTED_EDGE ( 'NONE', *, *, #16, .F. ) ;
#21568=VERTEX_POINT ( 'NONE', #10757 ) ;
#21639=AXIS2_PLACEMENT_3D ( 'NONE', #11876, #3637, #1944 ) ;
#21676=CARTESIAN_POINT ( 'NONE',  ( -0.7500000000000001110, 1.299038105676658450, 17.69999999999999929 ) ) ;
#21767=CARTESIAN_POINT ( 'NONE',  ( -0.7500000000000001110, 0.000000000000000000, 17.69999999999999929 ) ) ;
#21821=LINE ( 'NONE', #24152, #24667 ) ;
#21978=DIRECTION ( 'NONE',  ( 1.000000000000000000, 0.000000000000000000, 0.000000000000000000 ) ) ;
#22017=DIRECTION ( 'NONE',  ( 0.000000000000000000, 0.000000000000000000, 1.000000000000000000 ) ) ;
#22089=CARTESIAN_POINT ( 'NONE',  ( 0.7500000000000000000, 0.000000000000000000, 17.69999999999999929 ) ) ;
#22139=VECTOR ( 'NONE', #20872, 1000.000000000000000 ) ;
#22238=CARTESIAN_POINT ( 'NONE',  ( -0.7500000000000000000, -1.299038105676658450, 18.19999999999999929 ) ) ;
#22316=EDGE_CURVE ( 'NONE', #7827, #19442, #10021, .T. ) ;
#22344=CARTESIAN_POINT ( 'NONE',  ( 0.000000000000000000, 0.000000000000000000, 18.19999999999999929 ) ) ;
#22348=PRESENTATION_STYLE_ASSIGNMENT (( #15965 ) ) ;
#22359=LINE ( 'NONE', #4572, #1604 ) ;
#22485=CARTESIAN_POINT ( 'NONE',  ( -0.7500000000000001110, 20.00000000000000000, 17.69999999999999929 ) ) ;
#22565=ADVANCED_FACE ( 'NONE', ( #17223 ), #15736, .F. ) ;
#22573=DIRECTION ( 'NONE',  ( 0.000000000000000000, 0.000000000000000000, 1.000000000000000000 ) ) ;
#22579=EDGE_CURVE ( 'NONE', #19382, #25812, #25790, .T. ) ;
#22634=DIRECTION ( 'NONE',  ( -0.000000000000000000, -1.000000000000000000, 0.000000000000000000 ) ) ;
#22719=DIRECTION ( 'NONE',  ( 0.000000000000000000, 0.000000000000000000, 1.000000000000000000 ) ) ;
#22720=DIRECTION ( 'NONE',  ( 0.000000000000000000, 1.000000000000000000, 0.000000000000000000 ) ) ;
#22832=ORIENTED_EDGE ( 'NONE', *, *, #15885, .T. ) ;
#22839=FACE_OUTER_BOUND ( 'NONE', #13369, .T. ) ;
#22955=CARTESIAN_POINT ( 'NONE',  ( 1.500000000000000222, 0.000000000000000000, 17.69999999999999929 ) ) ;
#23008=CARTESIAN_POINT ( 'NONE',  ( -0.7500000000000000000, 0.000000000000000000, 17.69999999999999929 ) ) ;
#23079=CARTESIAN_POINT ( 'NONE',  ( -0.7500000000000001110, 1.299038105676658450, 17.69999999999999929 ) ) ;
#23092=CIRCLE ( 'NONE', #11807, 1.500000000000000222 ) ;
#23149=ORIENTED_EDGE ( 'NONE', *, *, #17150, .T. ) ;
#23151=DIRECTION ( 'NONE',  ( 0.000000000000000000, 0.000000000000000000, 1.000000000000000000 ) ) ;
#23164=DIRECTION ( 'NONE',  ( 1.000000000000000000, 0.000000000000000000, 0.000000000000000000 ) ) ;
#23184=EDGE_LOOP ( 'NONE', ( #18753, #3553, #24938, #15271 ) ) ;
#23252=PRODUCT_DEFINITION_CONTEXT ( 'detailed design', #15450, 'design' ) ;
#23330=ORIENTED_EDGE ( 'NONE', *, *, #4430, .T. ) ;
#23368=LINE ( 'NONE', #19439, #15484 ) ;
#23431=ORIENTED_EDGE ( 'NONE', *, *, #23598, .F. ) ;
#23479=EDGE_CURVE ( 'NONE', #5355, #15216, #13319, .T. ) ;
#23517=DIRECTION ( 'NONE',  ( -0.000000000000000000, -1.000000000000000000, 0.000000000000000000 ) ) ;
#23523=CARTESIAN_POINT ( 'NONE',  ( 0.7500000000000001110, 9.184850993605150903E-17, 18.19999999999999929 ) ) ;
#23596=ORIENTED_EDGE ( 'NONE', *, *, #4612, .T. ) ;
#23598=EDGE_CURVE ( 'NONE', #5872, #14663, #16781, .T. ) ;
#23607=( NAMED_UNIT ( * ) SI_UNIT ( $, .STERADIAN. ) SOLID_ANGLE_UNIT ( ) );
#23631=ORIENTED_EDGE ( 'NONE', *, *, #9563, .F. ) ;
#23662=DIRECTION ( 'NONE',  ( 0.000000000000000000, 0.000000000000000000, 1.000000000000000000 ) ) ;
#23664=CARTESIAN_POINT ( 'NONE',  ( 0.7500000000000000000, -1.299038105676658450, 18.19999999999999929 ) ) ;
#23697=EDGE_CURVE ( 'NONE', #25812, #25396, #12505, .T. ) ;
#23761=DIRECTION ( 'NONE',  ( 1.000000000000000000, 0.000000000000000000, 0.000000000000000000 ) ) ;
#23777=DIRECTION ( 'NONE',  ( -1.000000000000000000, 0.000000000000000000, 0.000000000000000000 ) ) ;
#23788=AXIS2_PLACEMENT_3D ( 'NONE', #11368, #11107, #15182 ) ;
#23791=MECHANICAL_DESIGN_GEOMETRIC_PRESENTATION_REPRESENTATION('',(#5405),#25865);
#23839=CARTESIAN_POINT ( 'NONE',  ( 0.7500000000000000000, -2.999999999999999556, 17.69999999999999929 ) ) ;
#24152=CARTESIAN_POINT ( 'NONE',  ( -0.7500000000000001110, 0.000000000000000000, 17.69999999999999929 ) ) ;
#24291=ORIENTED_EDGE ( 'NONE', *, *, #25796, .F. ) ;
#24355=EDGE_CURVE ( 'NONE', #3025, #24553, #7879, .T. ) ;
#24374=( GEOMETRIC_REPRESENTATION_CONTEXT ( 3 ) GLOBAL_UNCERTAINTY_ASSIGNED_CONTEXT ( ( #774 ) ) GLOBAL_UNIT_ASSIGNED_CONTEXT ( ( #11385, #11509, #3655 ) ) REPRESENTATION_CONTEXT ( 'NONE', 'WORKASPACE' ) );
#24393=CARTESIAN_POINT ( 'NONE',  ( 0.7500000000000000000, 0.000000000000000000, 18.19999999999999929 ) ) ;
#24550=ORIENTED_EDGE ( 'NONE', *, *, #11543, .F. ) ;
#24553=VERTEX_POINT ( 'NONE', #6175 ) ;
#24667=VECTOR ( 'NONE', #15799, 1000.000000000000000 ) ;
#24712=EDGE_CURVE ( 'NONE', #20366, #5872, #1552, .T. ) ;
#24800=CARTESIAN_POINT ( 'NONE',  ( 0.7500000000000000000, 0.000000000000000000, 17.69999999999999929 ) ) ;
#24875=AXIS2_PLACEMENT_3D ( 'NONE', #10722, #16511, #10996 ) ;
#24938=ORIENTED_EDGE ( 'NONE', *, *, #16, .T. ) ;
#25053=VECTOR ( 'NONE', #18021, 1000.000000000000000 ) ;
#25266=CARTESIAN_POINT ( 'NONE',  ( 0.7500000000000001110, 20.00000000000000000, 17.69999999999999929 ) ) ;
#25396=VERTEX_POINT ( 'NONE', #5774 ) ;
#25625=EDGE_LOOP ( 'NONE', ( #6742, #14277, #15080, #8916 ) ) ;
#25628=EDGE_LOOP ( 'NONE', ( #18559, #18844, #3846, #4550 ) ) ;
#25645=DIRECTION ( 'NONE',  ( 0.000000000000000000, 0.000000000000000000, 1.000000000000000000 ) ) ;
#25691=PLANE ( 'NONE',  #11398 ) ;
#25790=LINE ( 'NONE', #4913, #22139 ) ;
#25796=EDGE_CURVE ( 'NONE', #311, #25812, #18535, .T. ) ;
#25812=VERTEX_POINT ( 'NONE', #7073 ) ;
#25865=( GEOMETRIC_REPRESENTATION_CONTEXT ( 3 ) GLOBAL_UNCERTAINTY_ASSIGNED_CONTEXT ( ( #9131 ) ) GLOBAL_UNIT_ASSIGNED_CONTEXT ( ( #77, #19805, #23607 ) ) REPRESENTATION_CONTEXT ( 'NONE', 'WORKASPACE' ) );
#25901=COLOUR_RGB('Sky Blue',0.24,0.69,0.87);
#25902=FILL_AREA_STYLE_COLOUR('',#25901);
#25903=FILL_AREA_STYLE('',(#25902));
#25904=SURFACE_STYLE_FILL_AREA(#25903);
#25905=SURFACE_SIDE_STYLE('',(#25904));
#25906=SURFACE_STYLE_USAGE(.BOTH.,#25905);
#25907=PRESENTATION_STYLE_ASSIGNMENT((#25906));
ENDSEC;
END-ISO-10303-21;
